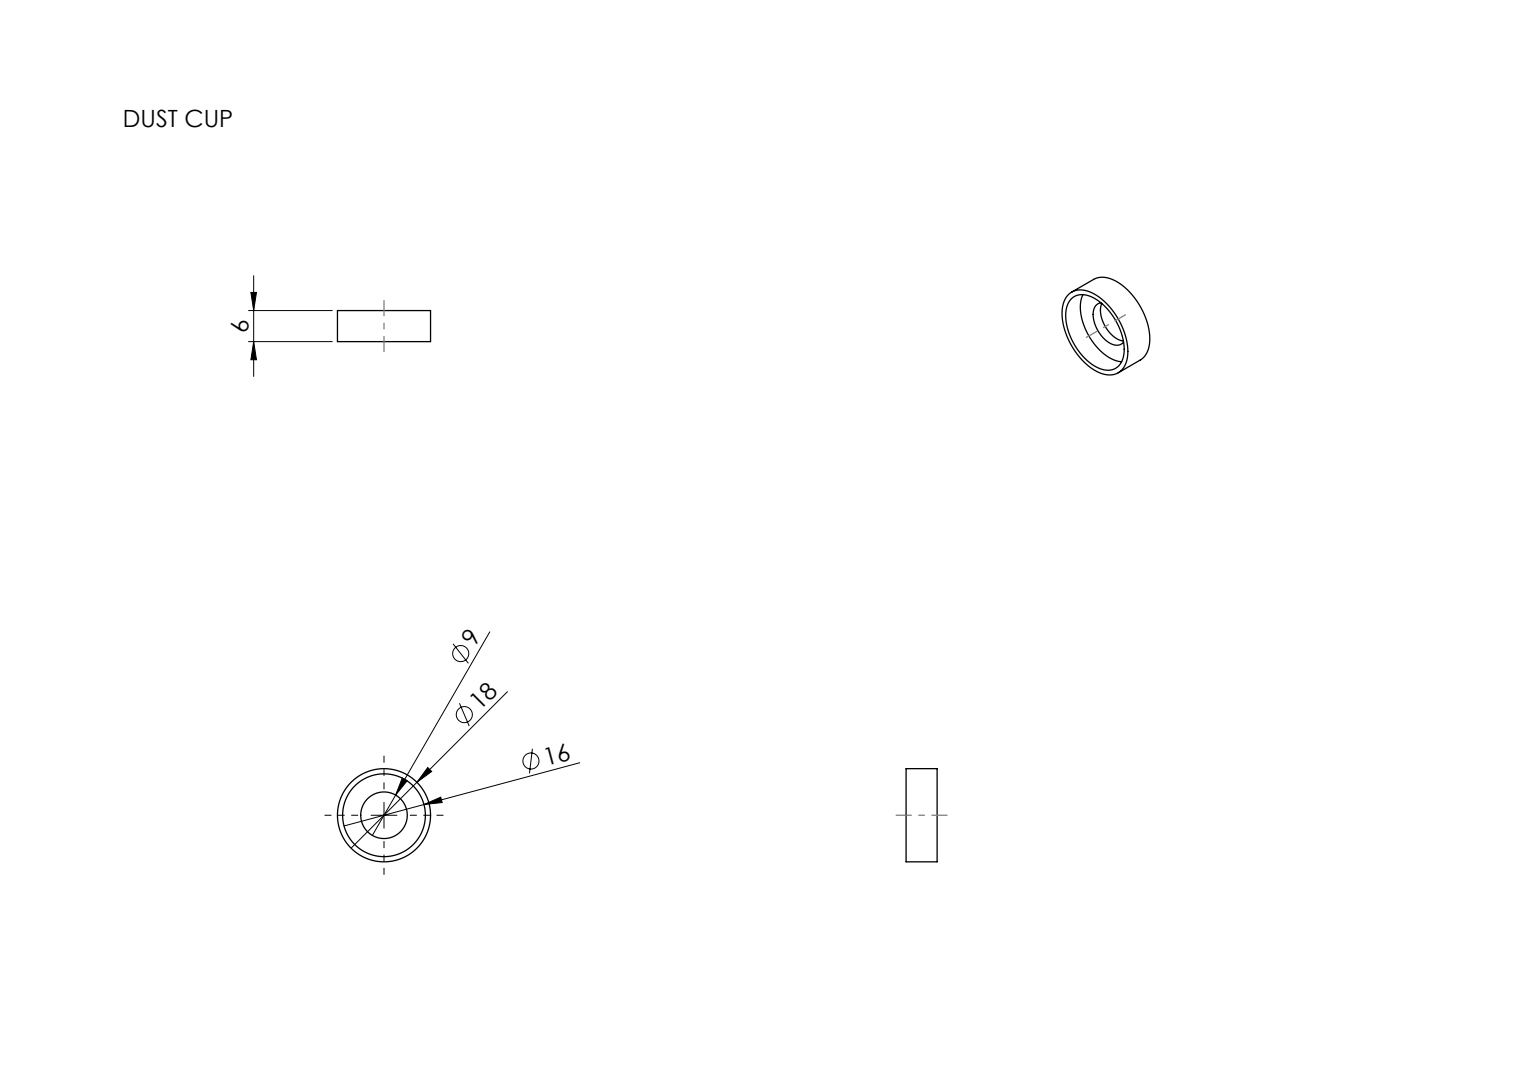
ISO-10303-21;
HEADER;
FILE_DESCRIPTION (('STEP AP214'),
    '1' );
FILE_NAME ('DUST CUP.step',
    '2026-10-08T05:56:58',
    ( '' ),
    ( '' ),
    'SwSTEP 2.0',
    'SolidWorks 2026',
    '' );
FILE_SCHEMA (( 'AUTOMOTIVE_DESIGN' ));
ENDSEC;

DATA;
#98=CARTESIAN_POINT ( 'NONE',  ( 0.000000000000000000, 0.000000000000000000, -35.00000000000000000 ) ) ;
#229=DIRECTION ( 'NONE',  ( -1.000000000000000000, 0.000000000000000000, 0.000000000000000000 ) ) ;
#249=SHAPE_DEFINITION_REPRESENTATION ( #10039, #10045 ) ;
#267=DIRECTION ( 'NONE',  ( 0.000000000000000000, 0.000000000000000000, 1.000000000000000000 ) ) ;
#450=ORIENTED_EDGE ( 'NONE', *, *, #18835, .T. ) ;
#457=FILL_AREA_STYLE_COLOUR ( '', #2219 ) ;
#510=DIRECTION ( 'NONE',  ( 0.000000000000000000, 0.000000000000000000, 1.000000000000000000 ) ) ;
#541=CARTESIAN_POINT ( 'NONE',  ( 0.000000000000000000, 0.000000000000000000, -33.00000000000000000 ) ) ;
#622=CARTESIAN_POINT ( 'NONE',  ( 0.000000000000000000, 0.000000000000000000, -33.00000000000000000 ) ) ;
#689=CIRCLE ( 'NONE', #18568, 9.000000000000000000 ) ;
#816=EDGE_CURVE ( 'NONE', #10379, #5629, #19401, .T. ) ;
#862=DIRECTION ( 'NONE',  ( -1.000000000000000000, 0.000000000000000000, 0.000000000000000000 ) ) ;
#944=SURFACE_SIDE_STYLE ('',( #18751 ) ) ;
#960=EDGE_LOOP ( 'NONE', ( #14125, #1610 ) ) ;
#981=SURFACE_STYLE_FILL_AREA ( #8681 ) ;
#1051=AXIS2_PLACEMENT_3D ( 'NONE', #541, #6513, #1831 ) ;
#1087=CARTESIAN_POINT ( 'NONE',  ( 0.000000000000000000, 0.000000000000000000, -35.00000000000000000 ) ) ;
#1112=CARTESIAN_POINT ( 'NONE',  ( 0.000000000000000000, 0.000000000000000000, -29.00000000000000000 ) ) ;
#1131=FACE_OUTER_BOUND ( 'NONE', #13815, .T. ) ;
#1185=UNCERTAINTY_MEASURE_WITH_UNIT (LENGTH_MEASURE( 1.000000000000000082E-05 ), #18893, 'distance_accuracy_value', 'NONE');
#1223=EDGE_LOOP ( 'NONE', ( #18942, #10771, #450, #12959 ) ) ;
#1262=AXIS2_PLACEMENT_3D ( 'NONE', #8364, #8469, #862 ) ;
#1265=( GEOMETRIC_REPRESENTATION_CONTEXT ( 3 ) GLOBAL_UNCERTAINTY_ASSIGNED_CONTEXT ( ( #3992 ) ) GLOBAL_UNIT_ASSIGNED_CONTEXT ( ( #19051, #2529, #14656 ) ) REPRESENTATION_CONTEXT ( 'NONE', 'WORKASPACE' ) );
#1266=DIRECTION ( 'NONE',  ( 0.000000000000000000, 0.000000000000000000, 1.000000000000000000 ) ) ;
#1331=DIRECTION ( 'NONE',  ( -1.000000000000000000, 0.000000000000000000, 0.000000000000000000 ) ) ;
#1417=ORIENTED_EDGE ( 'NONE', *, *, #6517, .F. ) ;
#1610=ORIENTED_EDGE ( 'NONE', *, *, #13748, .T. ) ;
#1662=ADVANCED_FACE ( 'NONE', ( #15826, #15725 ), #2016, .F. ) ;
#1675=CARTESIAN_POINT ( 'NONE',  ( 0.000000000000000000, 0.000000000000000000, -29.00000000000000000 ) ) ;
#1701=DIRECTION ( 'NONE',  ( 0.000000000000000000, 0.000000000000000000, -1.000000000000000000 ) ) ;
#1789=LINE ( 'NONE', #17293, #13177 ) ;
#1796=DIRECTION ( 'NONE',  ( -1.000000000000000000, 0.000000000000000000, 0.000000000000000000 ) ) ;
#1799=CARTESIAN_POINT ( 'NONE',  ( 0.000000000000000000, 0.000000000000000000, -35.00000000000000000 ) ) ;
#1831=DIRECTION ( 'NONE',  ( 1.000000000000000000, 0.000000000000000000, 0.000000000000000000 ) ) ;
#1913=DIRECTION ( 'NONE',  ( 0.000000000000000000, 0.000000000000000000, -1.000000000000000000 ) ) ;
#2016=PLANE ( 'NONE',  #16779 ) ;
#2198=LINE ( 'NONE', #6490, #3391 ) ;
#2219=COLOUR_RGB ( '', 0.66274510, 0.83137255, 0.94901961) ;
#2288=DIRECTION ( 'NONE',  ( -1.000000000000000000, 0.000000000000000000, 0.000000000000000000 ) ) ;
#2375=DIRECTION ( 'NONE',  ( -1.000000000000000000, 0.000000000000000000, -0.000000000000000000 ) ) ;
#2499=ORIENTED_EDGE ( 'NONE', *, *, #3937, .F. ) ;
#2529=( NAMED_UNIT ( * ) PLANE_ANGLE_UNIT ( ) SI_UNIT ( $, .RADIAN. ) );
#2571=CARTESIAN_POINT ( 'NONE',  ( 8.000000000000000000, 9.797174393178825657E-16, -33.00000000000000000 ) ) ;
#2617=CARTESIAN_POINT ( 'NONE',  ( 0.000000000000000000, 0.000000000000000000, -33.00000000000000000 ) ) ;
#2714=ORIENTED_EDGE ( 'NONE', *, *, #12629, .F. ) ;
#2725=CIRCLE ( 'NONE', #14572, 8.000000000000000000 ) ;
#2824=DIRECTION ( 'NONE',  ( 0.000000000000000000, 0.000000000000000000, -1.000000000000000000 ) ) ;
#2882=EDGE_LOOP ( 'NONE', ( #8062, #11799, #2714, #19306 ) ) ;
#2906=CIRCLE ( 'NONE', #4206, 8.000000000000000000 ) ;
#3132=EDGE_CURVE ( 'NONE', #5629, #6948, #13522, .T. ) ;
#3174=CYLINDRICAL_SURFACE ( 'NONE', #14334, 8.000000000000000000 ) ;
#3285=CARTESIAN_POINT ( 'NONE',  ( 9.000000000000000000, 1.102182119232617714E-15, -33.00000000000000000 ) ) ;
#3306=STYLED_ITEM ( 'NONE', ( #17790 ), #17347 ) ;
#3391=VECTOR ( 'NONE', #12519, 1000.000000000000000 ) ;
#3418=AXIS2_PLACEMENT_3D ( 'NONE', #1675, #267, #7564 ) ;
#3576=VERTEX_POINT ( 'NONE', #11230 ) ;
#3632=( GEOMETRIC_REPRESENTATION_CONTEXT ( 3 ) GLOBAL_UNCERTAINTY_ASSIGNED_CONTEXT ( ( #1185 ) ) GLOBAL_UNIT_ASSIGNED_CONTEXT ( ( #18893, #8584, #3986 ) ) REPRESENTATION_CONTEXT ( 'NONE', 'WORKASPACE' ) );
#3680=APPLICATION_CONTEXT ( 'automotive_design' ) ;
#3684=VECTOR ( 'NONE', #18301, 1000.000000000000000 ) ;
#3801=CIRCLE ( 'NONE', #8916, 9.000000000000000000 ) ;
#3808=DIRECTION ( 'NONE',  ( 0.000000000000000000, 0.000000000000000000, -1.000000000000000000 ) ) ;
#3881=SHAPE_REPRESENTATION_RELATIONSHIP ( 'NONE' , 'NONE' ,  #10045, #17347 ) ;
#3937=EDGE_CURVE ( 'NONE', #4109, #3576, #7249, .T. ) ;
#3986=( NAMED_UNIT ( * ) SI_UNIT ( $, .STERADIAN. ) SOLID_ANGLE_UNIT ( ) );
#3992=UNCERTAINTY_MEASURE_WITH_UNIT (LENGTH_MEASURE( 1.000000000000000082E-05 ), #19051, 'distance_accuracy_value', 'NONE');
#4086=SURFACE_SIDE_STYLE ('',( #981 ) ) ;
#4109=VERTEX_POINT ( 'NONE', #7947 ) ;
#4153=CYLINDRICAL_SURFACE ( 'NONE', #1262, 4.500000000000000000 ) ;
#4168=CARTESIAN_POINT ( 'NONE',  ( -8.000000000000000000, 0.000000000000000000, -33.00000000000000000 ) ) ;
#4206=AXIS2_PLACEMENT_3D ( 'NONE', #15959, #5628, #14461 ) ;
#4228=CYLINDRICAL_SURFACE ( 'NONE', #5317, 9.000000000000000000 ) ;
#4284=ORIENTED_EDGE ( 'NONE', *, *, #12312, .T. ) ;
#4399=CIRCLE ( 'NONE', #19093, 8.000000000000000000 ) ;
#4638=DIRECTION ( 'NONE',  ( -1.000000000000000000, 0.000000000000000000, 0.000000000000000000 ) ) ;
#4690=LINE ( 'NONE', #3285, #3684 ) ;
#4709=APPLICATION_CONTEXT ( 'automotive_design' ) ;
#4791=DIRECTION ( 'NONE',  ( -0.000000000000000000, -0.000000000000000000, -1.000000000000000000 ) ) ;
#4800=DIRECTION ( 'NONE',  ( -1.000000000000000000, 0.000000000000000000, 0.000000000000000000 ) ) ;
#4843=ORIENTED_EDGE ( 'NONE', *, *, #17415, .T. ) ;
#4996=DIRECTION ( 'NONE',  ( 0.000000000000000000, 0.000000000000000000, -1.000000000000000000 ) ) ;
#5012=ORIENTED_EDGE ( 'NONE', *, *, #9619, .F. ) ;
#5279=EDGE_CURVE ( 'NONE', #6013, #15601, #2725, .T. ) ;
#5307=LINE ( 'NONE', #6792, #10579 ) ;
#5317=AXIS2_PLACEMENT_3D ( 'NONE', #2617, #6112, #8731 ) ;
#5410=EDGE_LOOP ( 'NONE', ( #17654, #16795 ) ) ;
#5427=AXIS2_PLACEMENT_3D ( 'NONE', #7918, #8124, #229 ) ;
#5628=DIRECTION ( 'NONE',  ( 0.000000000000000000, 0.000000000000000000, 1.000000000000000000 ) ) ;
#5629=VERTEX_POINT ( 'NONE', #11625 ) ;
#5634=EDGE_LOOP ( 'NONE', ( #4284, #18522, #1417, #11359 ) ) ;
#5721=EDGE_LOOP ( 'NONE', ( #13208, #11260 ) ) ;
#5788=CARTESIAN_POINT ( 'NONE',  ( 8.000000000000000000, 9.797174393178825657E-16, -29.00000000000000000 ) ) ;
#5852=MECHANICAL_DESIGN_GEOMETRIC_PRESENTATION_REPRESENTATION('',(#3306),#9734);
#5890=EDGE_CURVE ( 'NONE', #12338, #6948, #2198, .T. ) ;
#5908=AXIS2_PLACEMENT_3D ( 'NONE', #10092, #6962, #2375 ) ;
#5930=CYLINDRICAL_SURFACE ( 'NONE', #14859, 4.500000000000000000 ) ;
#6013=VERTEX_POINT ( 'NONE', #11601 ) ;
#6064=FACE_OUTER_BOUND ( 'NONE', #960, .T. ) ;
#6112=DIRECTION ( 'NONE',  ( 0.000000000000000000, 0.000000000000000000, -1.000000000000000000 ) ) ;
#6194=DIRECTION ( 'NONE',  ( 1.000000000000000000, 0.000000000000000000, 0.000000000000000000 ) ) ;
#6230=DIRECTION ( 'NONE',  ( 1.000000000000000000, 0.000000000000000000, 0.000000000000000000 ) ) ;
#6350=ORIENTED_EDGE ( 'NONE', *, *, #12629, .T. ) ;
#6413=CIRCLE ( 'NONE', #1051, 8.000000000000000000 ) ;
#6480=CARTESIAN_POINT ( 'NONE',  ( 0.000000000000000000, 0.000000000000000000, -29.00000000000000000 ) ) ;
#6490=CARTESIAN_POINT ( 'NONE',  ( -4.500000000000000000, 0.000000000000000000, -33.00000000000000000 ) ) ;
#6513=DIRECTION ( 'NONE',  ( 0.000000000000000000, 0.000000000000000000, 1.000000000000000000 ) ) ;
#6517=EDGE_CURVE ( 'NONE', #8963, #12765, #2906, .T. ) ;
#6532=FILL_AREA_STYLE ('',( #457 ) ) ;
#6666=EDGE_CURVE ( 'NONE', #14571, #12630, #689, .T. ) ;
#6725=ORIENTED_EDGE ( 'NONE', *, *, #3132, .T. ) ;
#6792=CARTESIAN_POINT ( 'NONE',  ( -9.000000000000000000, 0.000000000000000000, -33.00000000000000000 ) ) ;
#6948=VERTEX_POINT ( 'NONE', #15736 ) ;
#6954=CIRCLE ( 'NONE', #8888, 9.000000000000000000 ) ;
#6962=DIRECTION ( 'NONE',  ( 0.000000000000000000, 0.000000000000000000, -1.000000000000000000 ) ) ;
#6971=CYLINDRICAL_SURFACE ( 'NONE', #15919, 8.000000000000000000 ) ;
#7021=PRESENTATION_STYLE_ASSIGNMENT (( #14459 ) ) ;
#7023=ORIENTED_EDGE ( 'NONE', *, *, #16502, .F. ) ;
#7107=EDGE_LOOP ( 'NONE', ( #6350, #14654 ) ) ;
#7249=CIRCLE ( 'NONE', #7894, 9.000000000000000000 ) ;
#7384=DIRECTION ( 'NONE',  ( 1.000000000000000000, 0.000000000000000000, 0.000000000000000000 ) ) ;
#7564=DIRECTION ( 'NONE',  ( 1.000000000000000000, 0.000000000000000000, -0.000000000000000000 ) ) ;
#7567=CARTESIAN_POINT ( 'NONE',  ( -9.000000000000000000, 0.000000000000000000, -35.00000000000000000 ) ) ;
#7602=ORIENTED_EDGE ( 'NONE', *, *, #816, .T. ) ;
#7730=DIRECTION ( 'NONE',  ( 0.000000000000000000, 0.000000000000000000, -1.000000000000000000 ) ) ;
#7773=DIRECTION ( 'NONE',  ( -1.000000000000000000, 0.000000000000000000, 0.000000000000000000 ) ) ;
#7793=CYLINDRICAL_SURFACE ( 'NONE', #10573, 9.000000000000000000 ) ;
#7894=AXIS2_PLACEMENT_3D ( 'NONE', #6480, #510, #6194 ) ;
#7918=CARTESIAN_POINT ( 'NONE',  ( 0.000000000000000000, 0.000000000000000000, -33.00000000000000000 ) ) ;
#7947=CARTESIAN_POINT ( 'NONE',  ( -9.000000000000000000, 0.000000000000000000, -29.00000000000000000 ) ) ;
#8062=ORIENTED_EDGE ( 'NONE', *, *, #13748, .F. ) ;
#8076=EDGE_CURVE ( 'NONE', #12765, #8963, #6413, .T. ) ;
#8091=PRODUCT_DEFINITION ( 'UNKNOWN', '', #9895, #14204 ) ;
#8124=DIRECTION ( 'NONE',  ( 0.000000000000000000, 0.000000000000000000, -1.000000000000000000 ) ) ;
#8364=CARTESIAN_POINT ( 'NONE',  ( 0.000000000000000000, 0.000000000000000000, -33.00000000000000000 ) ) ;
#8419=CARTESIAN_POINT ( 'NONE',  ( 4.500000000000000000, 5.510910596163088569E-16, -33.00000000000000000 ) ) ;
#8469=DIRECTION ( 'NONE',  ( 0.000000000000000000, 0.000000000000000000, -1.000000000000000000 ) ) ;
#8470=DIRECTION ( 'NONE',  ( 0.000000000000000000, 0.000000000000000000, -1.000000000000000000 ) ) ;
#8584=( NAMED_UNIT ( * ) PLANE_ANGLE_UNIT ( ) SI_UNIT ( $, .RADIAN. ) );
#8603=DIRECTION ( 'NONE',  ( 0.000000000000000000, 0.000000000000000000, -1.000000000000000000 ) ) ;
#8681=FILL_AREA_STYLE ('',( #11786 ) ) ;
#8731=DIRECTION ( 'NONE',  ( -1.000000000000000000, 0.000000000000000000, 0.000000000000000000 ) ) ;
#8850=AXIS2_PLACEMENT_3D ( 'NONE', #98, #1701, #17104 ) ;
#8887=DIRECTION ( 'NONE',  ( -1.000000000000000000, 0.000000000000000000, 0.000000000000000000 ) ) ;
#8888=AXIS2_PLACEMENT_3D ( 'NONE', #1087, #10295, #8887 ) ;
#8916=AXIS2_PLACEMENT_3D ( 'NONE', #11205, #12708, #12145 ) ;
#8947=FACE_OUTER_BOUND ( 'NONE', #14534, .T. ) ;
#8963=VERTEX_POINT ( 'NONE', #4168 ) ;
#9240=CARTESIAN_POINT ( 'NONE',  ( 0.000000000000000000, 0.000000000000000000, -35.00000000000000000 ) ) ;
#9285=DIRECTION ( 'NONE',  ( -0.000000000000000000, -0.000000000000000000, -1.000000000000000000 ) ) ;
#9349=ADVANCED_FACE ( 'NONE', ( #8947 ), #5930, .F. ) ;
#9619=EDGE_CURVE ( 'NONE', #3576, #14571, #4690, .T. ) ;
#9725=ADVANCED_FACE ( 'NONE', ( #9900, #11188 ), #13083, .T. ) ;
#9734=( GEOMETRIC_REPRESENTATION_CONTEXT ( 3 ) GLOBAL_UNCERTAINTY_ASSIGNED_CONTEXT ( ( #19002 ) ) GLOBAL_UNIT_ASSIGNED_CONTEXT ( ( #13091, #12997, #14790 ) ) REPRESENTATION_CONTEXT ( 'NONE', 'WORKASPACE' ) );
#9833=DIRECTION ( 'NONE',  ( 0.000000000000000000, 0.000000000000000000, 1.000000000000000000 ) ) ;
#9895=PRODUCT_DEFINITION_FORMATION_WITH_SPECIFIED_SOURCE ( 'ANY', '', #19444, .NOT_KNOWN. ) ;
#9900=FACE_BOUND ( 'NONE', #5410, .T. ) ;
#9908=SURFACE_STYLE_USAGE ( .BOTH. , #4086 ) ;
#10039=PRODUCT_DEFINITION_SHAPE ( 'NONE', 'NONE',  #8091 ) ;
#10045=SHAPE_REPRESENTATION ( 'DUST CUP', ( #16724 ), #3632 ) ;
#10092=CARTESIAN_POINT ( 'NONE',  ( 0.000000000000000000, 0.000000000000000000, -35.00000000000000000 ) ) ;
#10295=DIRECTION ( 'NONE',  ( 0.000000000000000000, 0.000000000000000000, -1.000000000000000000 ) ) ;
#10358=COLOUR_RGB ( '', 0.66274510, 0.83137255, 0.94901961) ;
#10379=VERTEX_POINT ( 'NONE', #10558 ) ;
#10492=ORIENTED_EDGE ( 'NONE', *, *, #12312, .F. ) ;
#10558=CARTESIAN_POINT ( 'NONE',  ( 4.500000000000000000, 5.510910596163088569E-16, -33.00000000000000000 ) ) ;
#10573=AXIS2_PLACEMENT_3D ( 'NONE', #13906, #16914, #1796 ) ;
#10575=CARTESIAN_POINT ( 'NONE',  ( 0.000000000000000000, 0.000000000000000000, -29.00000000000000000 ) ) ;
#10579=VECTOR ( 'NONE', #8603, 1000.000000000000000 ) ;
#10581=ADVANCED_FACE ( 'NONE', ( #1131 ), #4228, .T. ) ;
#10684=PLANE ( 'NONE',  #3418 ) ;
#10771=ORIENTED_EDGE ( 'NONE', *, *, #5279, .T. ) ;
#10883=CARTESIAN_POINT ( 'NONE',  ( 0.000000000000000000, 0.000000000000000000, -29.00000000000000000 ) ) ;
#10971=AXIS2_PLACEMENT_3D ( 'NONE', #1799, #4996, #4800 ) ;
#11001=FACE_OUTER_BOUND ( 'NONE', #2882, .T. ) ;
#11013=EDGE_CURVE ( 'NONE', #6013, #12765, #18112, .T. ) ;
#11061=ORIENTED_EDGE ( 'NONE', *, *, #5890, .T. ) ;
#11064=EDGE_CURVE ( 'NONE', #6948, #5629, #14915, .T. ) ;
#11129=ORIENTED_EDGE ( 'NONE', *, *, #11064, .T. ) ;
#11188=FACE_OUTER_BOUND ( 'NONE', #7107, .T. ) ;
#11205=CARTESIAN_POINT ( 'NONE',  ( 0.000000000000000000, 0.000000000000000000, -29.00000000000000000 ) ) ;
#11230=CARTESIAN_POINT ( 'NONE',  ( 9.000000000000000000, 1.102182119232617714E-15, -29.00000000000000000 ) ) ;
#11260=ORIENTED_EDGE ( 'NONE', *, *, #8076, .T. ) ;
#11359=ORIENTED_EDGE ( 'NONE', *, *, #18835, .F. ) ;
#11405=VECTOR ( 'NONE', #14910, 1000.000000000000000 ) ;
#11509=ADVANCED_FACE ( 'NONE', ( #6064, #18573 ), #10684, .T. ) ;
#11517=CARTESIAN_POINT ( 'NONE',  ( -8.000000000000000000, 0.000000000000000000, -29.00000000000000000 ) ) ;
#11601=CARTESIAN_POINT ( 'NONE',  ( 8.000000000000000000, 9.797174393178825657E-16, -29.00000000000000000 ) ) ;
#11624=VECTOR ( 'NONE', #3808, 1000.000000000000000 ) ;
#11625=CARTESIAN_POINT ( 'NONE',  ( 4.500000000000000000, 5.510910596163088569E-16, -35.00000000000000000 ) ) ;
#11786=FILL_AREA_STYLE_COLOUR ( '', #10358 ) ;
#11799=ORIENTED_EDGE ( 'NONE', *, *, #9619, .T. ) ;
#11802=STYLED_ITEM ( 'NONE', ( #7021 ), #16178 ) ;
#11933=ORIENTED_EDGE ( 'NONE', *, *, #5890, .F. ) ;
#12140=EDGE_LOOP ( 'NONE', ( #17665, #12814, #11061, #11129 ) ) ;
#12145=DIRECTION ( 'NONE',  ( 1.000000000000000000, 0.000000000000000000, 0.000000000000000000 ) ) ;
#12172=DIRECTION ( 'NONE',  ( 1.000000000000000000, 0.000000000000000000, 0.000000000000000000 ) ) ;
#12312=EDGE_CURVE ( 'NONE', #15601, #6013, #4399, .T. ) ;
#12338=VERTEX_POINT ( 'NONE', #19410 ) ;
#12519=DIRECTION ( 'NONE',  ( 0.000000000000000000, 0.000000000000000000, -1.000000000000000000 ) ) ;
#12582=ADVANCED_FACE ( 'NONE', ( #15802 ), #6971, .F. ) ;
#12629=EDGE_CURVE ( 'NONE', #12630, #14571, #6954, .T. ) ;
#12630=VERTEX_POINT ( 'NONE', #7567 ) ;
#12708=DIRECTION ( 'NONE',  ( 0.000000000000000000, 0.000000000000000000, 1.000000000000000000 ) ) ;
#12743=ORIENTED_EDGE ( 'NONE', *, *, #6666, .F. ) ;
#12765=VERTEX_POINT ( 'NONE', #2571 ) ;
#12814=ORIENTED_EDGE ( 'NONE', *, *, #19472, .F. ) ;
#12864=CIRCLE ( 'NONE', #19562, 4.500000000000000000 ) ;
#12916=ADVANCED_FACE ( 'NONE', ( #16893 ), #3174, .F. ) ;
#12959=ORIENTED_EDGE ( 'NONE', *, *, #8076, .F. ) ;
#12997=( NAMED_UNIT ( * ) PLANE_ANGLE_UNIT ( ) SI_UNIT ( $, .RADIAN. ) );
#13083=PLANE ( 'NONE',  #5908 ) ;
#13091=( LENGTH_UNIT ( ) NAMED_UNIT ( * ) SI_UNIT ( .MILLI., .METRE. ) );
#13177=VECTOR ( 'NONE', #4791, 1000.000000000000000 ) ;
#13208=ORIENTED_EDGE ( 'NONE', *, *, #6517, .T. ) ;
#13367=ORIENTED_EDGE ( 'NONE', *, *, #5279, .F. ) ;
#13522=CIRCLE ( 'NONE', #10971, 4.500000000000000000 ) ;
#13748=EDGE_CURVE ( 'NONE', #3576, #4109, #3801, .T. ) ;
#13815=EDGE_LOOP ( 'NONE', ( #5012, #2499, #4843, #12743 ) ) ;
#13906=CARTESIAN_POINT ( 'NONE',  ( 0.000000000000000000, 0.000000000000000000, -33.00000000000000000 ) ) ;
#13968=ADVANCED_FACE ( 'NONE', ( #16174 ), #4153, .F. ) ;
#14125=ORIENTED_EDGE ( 'NONE', *, *, #3937, .T. ) ;
#14204=PRODUCT_DEFINITION_CONTEXT ( 'detailed design', #4709, 'design' ) ;
#14334=AXIS2_PLACEMENT_3D ( 'NONE', #10883, #9285, #7773 ) ;
#14459=SURFACE_STYLE_USAGE ( .BOTH. , #944 ) ;
#14461=DIRECTION ( 'NONE',  ( 1.000000000000000000, 0.000000000000000000, 0.000000000000000000 ) ) ;
#14534=EDGE_LOOP ( 'NONE', ( #7023, #7602, #6725, #11933 ) ) ;
#14571=VERTEX_POINT ( 'NONE', #19476 ) ;
#14572=AXIS2_PLACEMENT_3D ( 'NONE', #10575, #1266, #12172 ) ;
#14654=ORIENTED_EDGE ( 'NONE', *, *, #6666, .T. ) ;
#14656=( NAMED_UNIT ( * ) SI_UNIT ( $, .STERADIAN. ) SOLID_ANGLE_UNIT ( ) );
#14693=CIRCLE ( 'NONE', #5427, 4.500000000000000000 ) ;
#14790=( NAMED_UNIT ( * ) SI_UNIT ( $, .STERADIAN. ) SOLID_ANGLE_UNIT ( ) );
#14859=AXIS2_PLACEMENT_3D ( 'NONE', #15049, #7730, #4638 ) ;
#14910=DIRECTION ( 'NONE',  ( -0.000000000000000000, -0.000000000000000000, -1.000000000000000000 ) ) ;
#14915=CIRCLE ( 'NONE', #8850, 4.500000000000000000 ) ;
#15049=CARTESIAN_POINT ( 'NONE',  ( 0.000000000000000000, 0.000000000000000000, -33.00000000000000000 ) ) ;
#15463=PRODUCT_CONTEXT ( 'NONE', #3680, 'mechanical' ) ;
#15601=VERTEX_POINT ( 'NONE', #11517 ) ;
#15725=FACE_OUTER_BOUND ( 'NONE', #5721, .T. ) ;
#15736=CARTESIAN_POINT ( 'NONE',  ( -4.500000000000000000, 0.000000000000000000, -35.00000000000000000 ) ) ;
#15802=FACE_OUTER_BOUND ( 'NONE', #5634, .T. ) ;
#15826=FACE_BOUND ( 'NONE', #18300, .T. ) ;
#15860=ADVANCED_FACE ( 'NONE', ( #11001 ), #7793, .T. ) ;
#15919=AXIS2_PLACEMENT_3D ( 'NONE', #19285, #17500, #2288 ) ;
#15959=CARTESIAN_POINT ( 'NONE',  ( 0.000000000000000000, 0.000000000000000000, -33.00000000000000000 ) ) ;
#16050=ORIENTED_EDGE ( 'NONE', *, *, #16502, .T. ) ;
#16077=DIRECTION ( 'NONE',  ( -1.000000000000000000, 0.000000000000000000, 0.000000000000000000 ) ) ;
#16174=FACE_OUTER_BOUND ( 'NONE', #12140, .T. ) ;
#16178=MANIFOLD_SOLID_BREP ( 'Extrude-Thin1', #17382 ) ;
#16502=EDGE_CURVE ( 'NONE', #10379, #12338, #14693, .T. ) ;
#16719=DIRECTION ( 'NONE',  ( 0.000000000000000000, 0.000000000000000000, 1.000000000000000000 ) ) ;
#16724=AXIS2_PLACEMENT_3D ( 'NONE', #17428, #9833, #6230 ) ;
#16779=AXIS2_PLACEMENT_3D ( 'NONE', #622, #1913, #18624 ) ;
#16795=ORIENTED_EDGE ( 'NONE', *, *, #3132, .F. ) ;
#16893=FACE_OUTER_BOUND ( 'NONE', #1223, .T. ) ;
#16914=DIRECTION ( 'NONE',  ( 0.000000000000000000, 0.000000000000000000, -1.000000000000000000 ) ) ;
#17104=DIRECTION ( 'NONE',  ( -1.000000000000000000, 0.000000000000000000, 0.000000000000000000 ) ) ;
#17293=CARTESIAN_POINT ( 'NONE',  ( -8.000000000000000000, 0.000000000000000000, -29.00000000000000000 ) ) ;
#17347=ADVANCED_BREP_SHAPE_REPRESENTATION ( '', ( #16178, #16724 ), #3632 ) ;
#17382=CLOSED_SHELL ( 'NONE', ( #12582, #9349, #15860, #1662, #10581, #9725, #13968, #11509, #12916 ) ) ;
#17415=EDGE_CURVE ( 'NONE', #4109, #12630, #5307, .T. ) ;
#17428=CARTESIAN_POINT ( 'NONE',  ( 0.000000000000000000, 0.000000000000000000, 0.000000000000000000 ) ) ;
#17471=CARTESIAN_POINT ( 'NONE',  ( 0.000000000000000000, 0.000000000000000000, -33.00000000000000000 ) ) ;
#17500=DIRECTION ( 'NONE',  ( -0.000000000000000000, -0.000000000000000000, -1.000000000000000000 ) ) ;
#17654=ORIENTED_EDGE ( 'NONE', *, *, #11064, .F. ) ;
#17665=ORIENTED_EDGE ( 'NONE', *, *, #816, .F. ) ;
#17770=EDGE_LOOP ( 'NONE', ( #10492, #13367 ) ) ;
#17778=ORIENTED_EDGE ( 'NONE', *, *, #19472, .T. ) ;
#17790=PRESENTATION_STYLE_ASSIGNMENT (( #9908 ) ) ;
#17873=MECHANICAL_DESIGN_GEOMETRIC_PRESENTATION_REPRESENTATION('',(#11802),#1265);
#18112=LINE ( 'NONE', #5788, #11405 ) ;
#18300=EDGE_LOOP ( 'NONE', ( #17778, #16050 ) ) ;
#18301=DIRECTION ( 'NONE',  ( 0.000000000000000000, 0.000000000000000000, -1.000000000000000000 ) ) ;
#18522=ORIENTED_EDGE ( 'NONE', *, *, #11013, .T. ) ;
#18568=AXIS2_PLACEMENT_3D ( 'NONE', #9240, #2824, #1331 ) ;
#18573=FACE_BOUND ( 'NONE', #17770, .T. ) ;
#18624=DIRECTION ( 'NONE',  ( -1.000000000000000000, 0.000000000000000000, -0.000000000000000000 ) ) ;
#18751=SURFACE_STYLE_FILL_AREA ( #6532 ) ;
#18835=EDGE_CURVE ( 'NONE', #15601, #8963, #1789, .T. ) ;
#18893=( LENGTH_UNIT ( ) NAMED_UNIT ( * ) SI_UNIT ( .MILLI., .METRE. ) );
#18942=ORIENTED_EDGE ( 'NONE', *, *, #11013, .F. ) ;
#19002=UNCERTAINTY_MEASURE_WITH_UNIT (LENGTH_MEASURE( 1.000000000000000082E-05 ), #13091, 'distance_accuracy_value', 'NONE');
#19051=( LENGTH_UNIT ( ) NAMED_UNIT ( * ) SI_UNIT ( .MILLI., .METRE. ) );
#19093=AXIS2_PLACEMENT_3D ( 'NONE', #1112, #16719, #7384 ) ;
#19285=CARTESIAN_POINT ( 'NONE',  ( 0.000000000000000000, 0.000000000000000000, -29.00000000000000000 ) ) ;
#19306=ORIENTED_EDGE ( 'NONE', *, *, #17415, .F. ) ;
#19401=LINE ( 'NONE', #8419, #11624 ) ;
#19410=CARTESIAN_POINT ( 'NONE',  ( -4.500000000000000000, 0.000000000000000000, -33.00000000000000000 ) ) ;
#19444=PRODUCT ( 'DUST CUP', 'DUST CUP', '', ( #15463 ) ) ;
#19472=EDGE_CURVE ( 'NONE', #12338, #10379, #12864, .T. ) ;
#19476=CARTESIAN_POINT ( 'NONE',  ( 9.000000000000000000, 1.102182119232617714E-15, -35.00000000000000000 ) ) ;
#19562=AXIS2_PLACEMENT_3D ( 'NONE', #17471, #8470, #16077 ) ;
ENDSEC;
END-ISO-10303-21;
